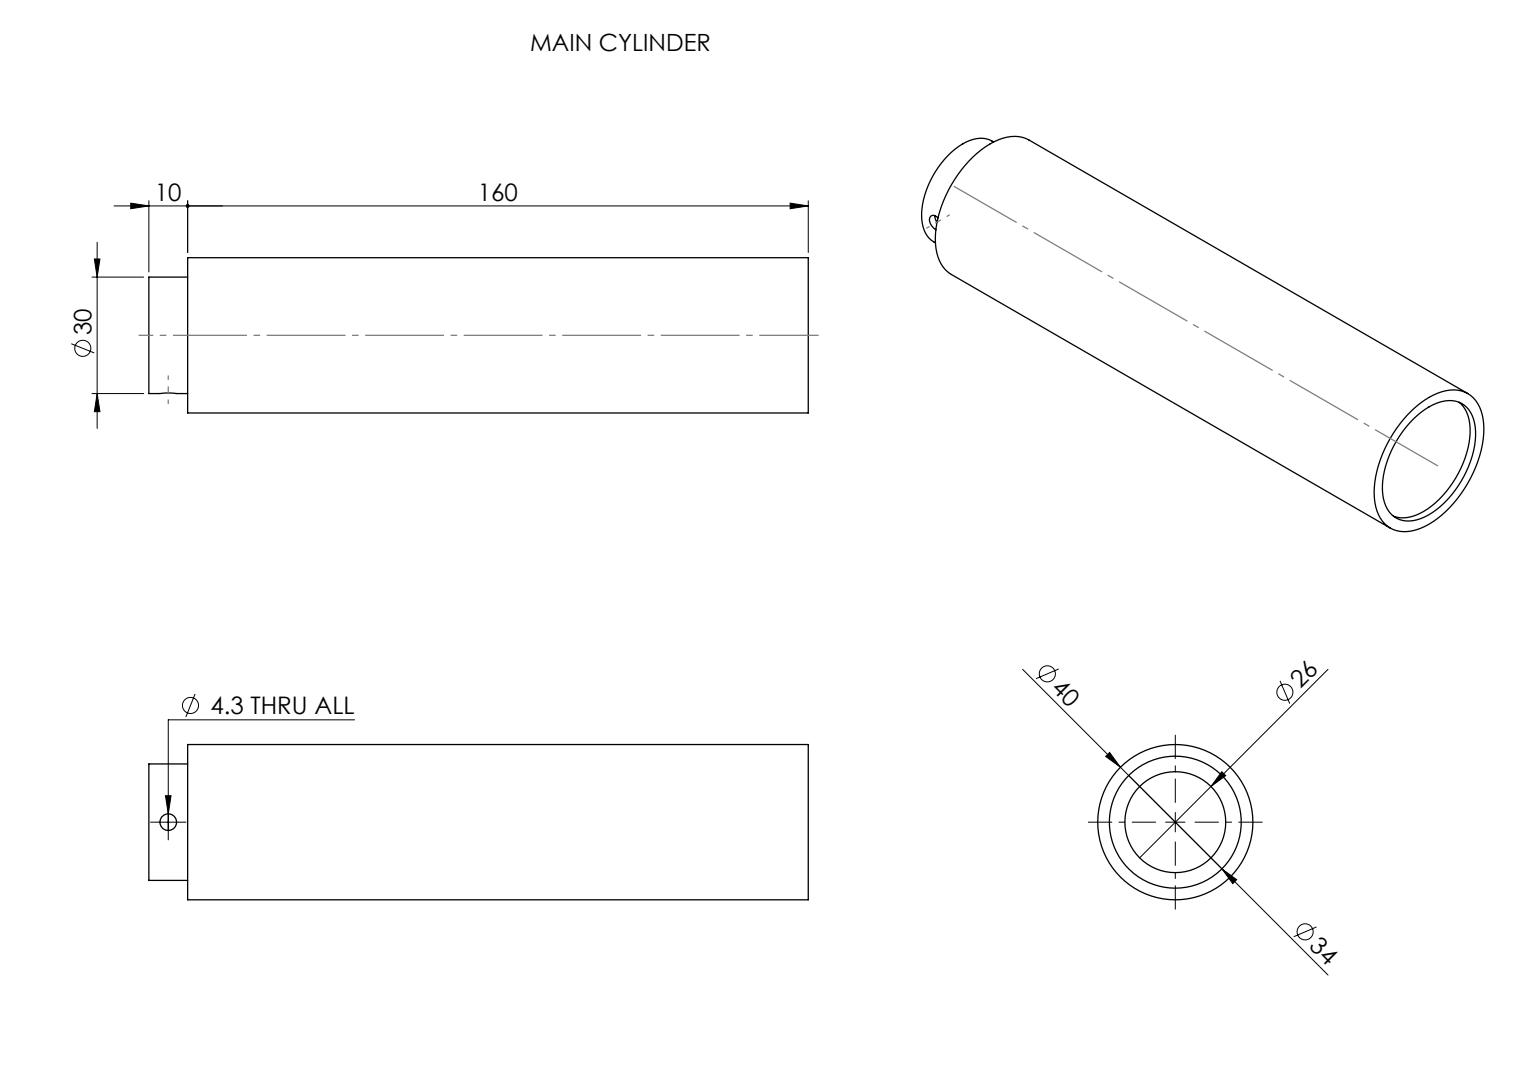
ISO-10303-21;
HEADER;
FILE_DESCRIPTION (('STEP AP214'),
    '1' );
FILE_NAME ('main cylinder.step',
    '2026-10-08T13:22:57',
    ( '' ),
    ( '' ),
    'SwSTEP 2.0',
    'SolidWorks 2026',
    '' );
FILE_SCHEMA (( 'AUTOMOTIVE_DESIGN' ));
ENDSEC;

DATA;
#66=DIRECTION ( 'NONE',  ( 1.000000000000000000, 4.755747939841215952E-17, -0.000000000000000000 ) ) ;
#75=CARTESIAN_POINT ( 'NONE',  ( -163.1352118936811451, 1.079191317860220156, 12.95565487998667820 ) ) ;
#78=ORIENTED_EDGE ( 'NONE', *, *, #9774, .F. ) ;
#81=DIRECTION ( 'NONE',  ( -4.755747939841216568E-17, 1.000000000000000000, 0.000000000000000000 ) ) ;
#98=CARTESIAN_POINT ( 'NONE',  ( -160.0000000000000284, 19.99999999999999289, 0.000000000000000000 ) ) ;
#120=CARTESIAN_POINT ( 'NONE',  ( -167.0926989554971556, -0.5670040589733402747, 14.99151548021192148 ) ) ;
#123=CARTESIAN_POINT ( 'NONE',  ( -166.9317395015584680, 0.9543248124665052456, 12.96558013998003922 ) ) ;
#132=ADVANCED_FACE ( 'NONE', ( #2160 ), #9918, .F. ) ;
#170=CARTESIAN_POINT ( 'NONE',  ( -165.9524913265358350, -1.932636693197999911, 14.87507538773749438 ) ) ;
#175=CARTESIAN_POINT ( 'NONE',  ( -166.3219090446497432, 1.718560695228406932, 12.88744630017030168 ) ) ;
#222=CARTESIAN_POINT ( 'NONE',  ( -8.084771497730057628E-16, 16.99999999999997868, 0.000000000000000000 ) ) ;
#225=CARTESIAN_POINT ( 'NONE',  ( -164.3051146695663363, -2.039487319166105372, 14.86080315614530534 ) ) ;
#228=CARTESIAN_POINT ( 'NONE',  ( -164.8603154174794270, 2.150053139255677870, 12.82096999065581322 ) ) ;
#239=DIRECTION ( 'NONE',  ( -4.755747939841215952E-17, 1.000000000000000000, 0.000000000000000000 ) ) ;
#245=CARTESIAN_POINT ( 'NONE',  ( 0.000000000000000000, 0.000000000000000000, 0.000000000000000000 ) ) ;
#257=APPLICATION_CONTEXT ( 'automotive_design' ) ;
#261=EDGE_LOOP ( 'NONE', ( #862, #304 ) ) ;
#274=DIRECTION ( 'NONE',  ( 0.000000000000000000, 1.000000000000000000, 0.000000000000000000 ) ) ;
#277=CARTESIAN_POINT ( 'NONE',  ( -164.4415472335243180, -2.080930162503950687, 14.85498226103907626 ) ) ;
#291=FACE_BOUND ( 'NONE', #7704, .T. ) ;
#297=DIRECTION ( 'NONE',  ( 1.000000000000000000, 4.755747939841215952E-17, -0.000000000000000000 ) ) ;
#302=ORIENTED_EDGE ( 'NONE', *, *, #7014, .T. ) ;
#304=ORIENTED_EDGE ( 'NONE', *, *, #4917, .T. ) ;
#308=PRODUCT ( 'main cylinder', 'main cylinder', '', ( #3194 ) ) ;
#311=ORIENTED_EDGE ( 'NONE', *, *, #4917, .F. ) ;
#314=DIRECTION ( 'NONE',  ( 0.000000000000000000, 1.000000000000000000, 0.000000000000000000 ) ) ;
#326=CARTESIAN_POINT ( 'NONE',  ( -164.0447505768503618, -1.931287831231678132, 14.87525146959452371 ) ) ;
#335=EDGE_LOOP ( 'NONE', ( #1912, #1497, #4062, #8563 ) ) ;
#345=VECTOR ( 'NONE', #3233, 1000.000000000000000 ) ;
#349=( NAMED_UNIT ( * ) SI_UNIT ( $, .STERADIAN. ) SOLID_ANGLE_UNIT ( ) );
#386=VECTOR ( 'NONE', #1036, 1000.000000000000000 ) ;
#401=ADVANCED_FACE ( 'NONE', ( #10107 ), #1214, .F. ) ;
#434=CARTESIAN_POINT ( 'NONE',  ( -162.8500000000000512, -5.808233104102145682E-15, 0.000000000000000000 ) ) ;
#443=FILL_AREA_STYLE ('',( #9851 ) ) ;
#468=DIRECTION ( 'NONE',  ( 1.000000000000000000, 4.755747939841215952E-17, -0.000000000000000000 ) ) ;
#485=ORIENTED_EDGE ( 'NONE', *, *, #7973, .F. ) ;
#507=MECHANICAL_DESIGN_GEOMETRIC_PRESENTATION_REPRESENTATION('',(#4963),#2980);
#517=ORIENTED_EDGE ( 'NONE', *, *, #4719, .F. ) ;
#544=CARTESIAN_POINT ( 'NONE',  ( -2.000000000000000888, -18.00000000000000355, 2.204364238465235822E-15 ) ) ;
#557=VERTEX_POINT ( 'NONE', #5547 ) ;
#594=VERTEX_POINT ( 'NONE', #10205 ) ;
#639=DIRECTION ( 'NONE',  ( 4.755747939841215952E-17, -1.000000000000000000, 0.000000000000000000 ) ) ;
#647=ORIENTED_EDGE ( 'NONE', *, *, #769, .T. ) ;
#664=EDGE_LOOP ( 'NONE', ( #485, #1187 ) ) ;
#675=AXIS2_PLACEMENT_3D ( 'NONE', #8769, #866, #81 ) ;
#679=CIRCLE ( 'NONE', #4292, 15.00000000000000000 ) ;
#699=CARTESIAN_POINT ( 'NONE',  ( -166.0761157388880918, -1.866610437352971719, 12.86553408738820714 ) ) ;
#714=DIRECTION ( 'NONE',  ( 1.000000000000000000, 4.755747939841215952E-17, -0.000000000000000000 ) ) ;
#715=ORIENTED_EDGE ( 'NONE', *, *, #7105, .T. ) ;
#755=EDGE_CURVE ( 'NONE', #7104, #6156, #3859, .T. ) ;
#769=EDGE_CURVE ( 'NONE', #9409, #594, #5277, .T. ) ;
#789=SHAPE_REPRESENTATION ( 'main cylinder', ( #3995 ), #10094 ) ;
#792=CARTESIAN_POINT ( 'NONE',  ( -166.4202771397491176, -1.620148664718404685, 12.89903195109847545 ) ) ;
#810=CARTESIAN_POINT ( 'NONE',  ( 0.000000000000000000, 5.592146987065130084E-32, 0.000000000000000000 ) ) ;
#812=CARTESIAN_POINT ( 'NONE',  ( -170.0000000000000284, -13.00000000000001066, 1.592040838891559687E-15 ) ) ;
#862=ORIENTED_EDGE ( 'NONE', *, *, #8540, .T. ) ;
#866=DIRECTION ( 'NONE',  ( 1.000000000000000000, 4.755747939841215952E-17, -0.000000000000000000 ) ) ;
#868=CIRCLE ( 'NONE', #8955, 18.00000000000000355 ) ;
#890=VECTOR ( 'NONE', #2246, 1000.000000000000000 ) ;
#913=VERTEX_POINT ( 'NONE', #98 ) ;
#955=CARTESIAN_POINT ( 'NONE',  ( -164.8564506259586153, -2.149904186608886381, 14.84513091884608649 ) ) ;
#970=PRODUCT_DEFINITION_FORMATION_WITH_SPECIFIED_SOURCE ( 'ANY', '', #308, .NOT_KNOWN. ) ;
#1003=CARTESIAN_POINT ( 'NONE',  ( -163.1340397805202542, -1.077317138390382345, 14.96172600814708353 ) ) ;
#1005=AXIS2_PLACEMENT_3D ( 'NONE', #7687, #7878, #1431 ) ;
#1035=VERTEX_POINT ( 'NONE', #4037 ) ;
#1036=DIRECTION ( 'NONE',  ( 1.000000000000000000, 4.755747939841215952E-17, -0.000000000000000000 ) ) ;
#1064=CARTESIAN_POINT ( 'NONE',  ( -162.8500000000000512, -5.808233196467851957E-15, 13.00000000000000178 ) ) ;
#1109=CARTESIAN_POINT ( 'NONE',  ( -165.5555415711045839, -2.081714733226260439, 14.85487199390593283 ) ) ;
#1131=EDGE_LOOP ( 'NONE', ( #4189, #4952 ) ) ;
#1146=ADVANCED_FACE ( 'NONE', ( #3187 ), #8668, .F. ) ;
#1156=CARTESIAN_POINT ( 'NONE',  ( -163.9215233434256618, 1.865203048549891163, 14.88378837804381583 ) ) ;
#1172=( LENGTH_UNIT ( ) NAMED_UNIT ( * ) SI_UNIT ( .MILLI., .METRE. ) );
#1180=AXIS2_PLACEMENT_3D ( 'NONE', #4946, #297, #8301 ) ;
#1187=ORIENTED_EDGE ( 'NONE', *, *, #8517, .F. ) ;
#1193=CARTESIAN_POINT ( 'NONE',  ( -160.0000000000000284, -7.609196703745946707E-15, 0.000000000000000000 ) ) ;
#1214=CYLINDRICAL_SURFACE ( 'NONE', #2628, 13.00000000000000178 ) ;
#1252=DIRECTION ( 'NONE',  ( -4.818676322157796389E-17, 1.000000000000000000, 0.000000000000000000 ) ) ;
#1259=CYLINDRICAL_SURFACE ( 'NONE', #4163, 15.00000000000000000 ) ;
#1306=CARTESIAN_POINT ( 'NONE',  ( -163.0677270160816192, 0.9532360713981521405, 14.97024790547416373 ) ) ;
#1330=FACE_BOUND ( 'NONE', #2547, .T. ) ;
#1341=AXIS2_PLACEMENT_3D ( 'NONE', #3965, #8237, #9078 ) ;
#1343=EDGE_CURVE ( 'NONE', #8824, #4150, #5768, .T. ) ;
#1345=ORIENTED_EDGE ( 'NONE', *, *, #5402, .F. ) ;
#1364=CARTESIAN_POINT ( 'NONE',  ( -164.8566404013504041, -2.149912913094245148, 12.82099350572476837 ) ) ;
#1399=VECTOR ( 'NONE', #8490, 1000.000000000000000 ) ;
#1400=EDGE_LOOP ( 'NONE', ( #5003, #9129, #5622, #9488 ) ) ;
#1431=DIRECTION ( 'NONE',  ( -4.755747939841215952E-17, 1.000000000000000000, 0.000000000000000000 ) ) ;
#1436=VERTEX_POINT ( 'NONE', #7998 ) ;
#1451=ORIENTED_EDGE ( 'NONE', *, *, #7973, .T. ) ;
#1468=CARTESIAN_POINT ( 'NONE',  ( -165.1407354622004391, -2.150086286197278707, 12.82096443211790060 ) ) ;
#1472=ORIENTED_EDGE ( 'NONE', *, *, #9157, .F. ) ;
#1497=ORIENTED_EDGE ( 'NONE', *, *, #1343, .F. ) ;
#1513=ORIENTED_EDGE ( 'NONE', *, *, #7634, .T. ) ;
#1521=CARTESIAN_POINT ( 'NONE',  ( -163.0673332015201709, -0.9523206289711777517, 12.96571997834879397 ) ) ;
#1565=ORIENTED_EDGE ( 'NONE', *, *, #2537, .F. ) ;
#1573=CARTESIAN_POINT ( 'NONE',  ( -163.3797476145753365, -1.420181920198508418, 12.92257903765585247 ) ) ;
#1586=CARTESIAN_POINT ( 'NONE',  ( -158.0000000000000284, -7.514081744949122117E-15, 0.000000000000000000 ) ) ;
#1596=SHAPE_DEFINITION_REPRESENTATION ( #1956, #789 ) ;
#1631=DIRECTION ( 'NONE',  ( 1.000000000000000000, 4.755747939841215952E-17, -0.000000000000000000 ) ) ;
#1663=ORIENTED_EDGE ( 'NONE', *, *, #6058, .F. ) ;
#1680=( GEOMETRIC_REPRESENTATION_CONTEXT ( 3 ) GLOBAL_UNCERTAINTY_ASSIGNED_CONTEXT ( ( #7319 ) ) GLOBAL_UNIT_ASSIGNED_CONTEXT ( ( #1172, #8987, #349 ) ) REPRESENTATION_CONTEXT ( 'NONE', 'WORKASPACE' ) );
#1687=CARTESIAN_POINT ( 'NONE',  ( -165.5651189253971722, 2.093213258176506386, 12.83083170865760181 ) ) ;
#1707=ORIENTED_EDGE ( 'NONE', *, *, #6644, .F. ) ;
#1716=AXIS2_PLACEMENT_3D ( 'NONE', #7873, #7733, #6362 ) ;
#1725=CIRCLE ( 'NONE', #5513, 13.00000000000000000 ) ;
#1731=CARTESIAN_POINT ( 'NONE',  ( -165.2804454449952516, -2.136238053246409141, 14.84712918936600623 ) ) ;
#1734=CARTESIAN_POINT ( 'NONE',  ( -160.0000000000000284, -7.609196703745946707E-15, 0.000000000000000000 ) ) ;
#1754=DIRECTION ( 'NONE',  ( 1.000000000000000000, 4.755747939841215952E-17, -0.000000000000000000 ) ) ;
#1760=ORIENTED_EDGE ( 'NONE', *, *, #4876, .T. ) ;
#1768=DIRECTION ( 'NONE',  ( -1.000000000000000000, -4.755747939841215952E-17, 0.000000000000000000 ) ) ;
#1779=DIRECTION ( 'NONE',  ( 0.000000000000000000, 1.000000000000000000, 0.000000000000000000 ) ) ;
#1784=ORIENTED_EDGE ( 'NONE', *, *, #755, .F. ) ;
#1789=DIRECTION ( 'NONE',  ( 1.000000000000000000, 4.755747939841215952E-17, -0.000000000000000000 ) ) ;
#1812=CYLINDRICAL_SURFACE ( 'NONE', #2046, 13.00000000000000178 ) ;
#1839=( LENGTH_UNIT ( ) NAMED_UNIT ( * ) SI_UNIT ( .MILLI., .METRE. ) );
#1844=UNCERTAINTY_MEASURE_WITH_UNIT (LENGTH_MEASURE( 1.000000000000000082E-05 ), #1839, 'distance_accuracy_value', 'NONE');
#1847=FILL_AREA_STYLE ('',( #5710 ) ) ;
#1882=CARTESIAN_POINT ( 'NONE',  ( -167.1500000000000341, -1.102909754258692077E-14, 15.00000000000000000 ) ) ;
#1885=CARTESIAN_POINT ( 'NONE',  ( -170.0000000000000284, 14.99999999999999289, 0.000000000000000000 ) ) ;
#1912=ORIENTED_EDGE ( 'NONE', *, *, #4905, .F. ) ;
#1918=DIRECTION ( 'NONE',  ( -5.102127870520027391E-17, 1.000000000000000000, 0.000000000000000000 ) ) ;
#1956=PRODUCT_DEFINITION_SHAPE ( 'NONE', 'NONE',  #4671 ) ;
#1979=CARTESIAN_POINT ( 'NONE',  ( -162.8500000000000512, -5.808233151972152598E-15, 15.00000000000000000 ) ) ;
#1987=DIRECTION ( 'NONE',  ( 1.000000000000000000, 4.755747939841215952E-17, -0.000000000000000000 ) ) ;
#1989=SURFACE_STYLE_FILL_AREA ( #443 ) ;
#1997=EDGE_CURVE ( 'NONE', #5632, #3401, #5774, .T. ) ;
#2038=PLANE ( 'NONE',  #5285 ) ;
#2041=UNCERTAINTY_MEASURE_WITH_UNIT (LENGTH_MEASURE( 1.000000000000000082E-05 ), #9661, 'distance_accuracy_value', 'NONE');
#2046=AXIS2_PLACEMENT_3D ( 'NONE', #8898, #2536, #8744 ) ;
#2074=EDGE_LOOP ( 'NONE', ( #5257, #2621, #7678, #7409 ) ) ;
#2081=CARTESIAN_POINT ( 'NONE',  ( -164.0471552234704689, 1.932476761857848668, 14.87509648533473516 ) ) ;
#2093=EDGE_CURVE ( 'NONE', #8307, #2751, #9346, .T. ) ;
#2106=FACE_OUTER_BOUND ( 'NONE', #8841, .T. ) ;
#2135=CARTESIAN_POINT ( 'NONE',  ( -165.6926619388180484, -2.040225341766198408, 12.83902055342544379 ) ) ;
#2158=ORIENTED_EDGE ( 'NONE', *, *, #7634, .F. ) ;
#2160=FACE_OUTER_BOUND ( 'NONE', #6889, .T. ) ;
#2171=EDGE_CURVE ( 'NONE', #6156, #1436, #3387, .T. ) ;
#2177=ORIENTED_EDGE ( 'NONE', *, *, #4861, .T. ) ;
#2192=CARTESIAN_POINT ( 'NONE',  ( -167.1500000000000341, -0.1422832181819098096, 13.00000000000000178 ) ) ;
#2246=DIRECTION ( 'NONE',  ( 1.000000000000000000, 4.755747939841215952E-17, -0.000000000000000000 ) ) ;
#2268=AXIS2_PLACEMENT_3D ( 'NONE', #2992, #6135, #9311 ) ;
#2292=CARTESIAN_POINT ( 'NONE',  ( -167.0388786721946701, -0.6964701277567462157, 12.98197609665553287 ) ) ;
#2298=CARTESIAN_POINT ( 'NONE',  ( 0.000000000000000000, 5.592146987065130084E-32, 0.000000000000000000 ) ) ;
#2312=DIRECTION ( 'NONE',  ( 0.000000000000000000, 1.000000000000000000, 0.000000000000000000 ) ) ;
#2340=CARTESIAN_POINT ( 'NONE',  ( -164.4413679183172121, -2.080883175690475539, 12.83240817167530246 ) ) ;
#2381=B_SPLINE_CURVE_WITH_KNOTS ( 'NONE', 3,
 ( #7253, #8759, #9543, #7306, #8820, #123, #4778, #3333, #2450, #175, #4058, #1687, #3228, #228, #6470, #9648, #5550, #3381, #8709, #5596, #5744, #4829, #7982, #75, #8079, #9693, #4205, #4157, #8913, #1064 ),
 .UNSPECIFIED., .F., .F.,
 ( 4, 2, 2, 2, 2, 2, 2, 2, 2, 2, 2, 2, 2, 2, 4 ),
 ( 5.712404575677604335E-19, 0.0004208408401708223071, 0.0008416816803416437469, 0.001262522520512465458, 0.001683363360683286626, 0.002525045041024870634, 0.003366726721366455292, 0.003787567561537246753, 0.004208408401708039516, 0.004629249241878830544, 0.005050090082049622439, 0.005470930922220414334, 0.005891771762391206230, 0.006312612602561998125, 0.006733453442732789153 ),
 .UNSPECIFIED. ) ;
#2402=CYLINDRICAL_SURFACE ( 'NONE', #8419, 18.00000000000000355 ) ;
#2450=CARTESIAN_POINT ( 'NONE',  ( -166.6189502573242578, 1.421653495296104408, 12.92241587668698166 ) ) ;
#2468=EDGE_LOOP ( 'NONE', ( #78, #6017, #4100, #7426 ) ) ;
#2470=LINE ( 'NONE', #5570, #8453 ) ;
#2499=CARTESIAN_POINT ( 'NONE',  ( -166.7173525949050088, -1.323475700837307700, 14.94282300546550069 ) ) ;
#2504=AXIS2_PLACEMENT_3D ( 'NONE', #2298, #2959, #5442 ) ;
#2507=EDGE_LOOP ( 'NONE', ( #9847, #7329 ) ) ;
#2532=ORIENTED_EDGE ( 'NONE', *, *, #8210, .F. ) ;
#2536=DIRECTION ( 'NONE',  ( 1.000000000000000000, 4.755747939841215952E-17, -0.000000000000000000 ) ) ;
#2537=EDGE_CURVE ( 'NONE', #594, #9409, #5452, .T. ) ;
#2547=EDGE_LOOP ( 'NONE', ( #3091, #8288 ) ) ;
#2551=CARTESIAN_POINT ( 'NONE',  ( -165.1406648078596220, -2.150094845865166082, 14.84510330590739180 ) ) ;
#2569=SURFACE_SIDE_STYLE ('',( #6482 ) ) ;
#2579=ADVANCED_FACE ( 'NONE', ( #5084 ), #8235, .T. ) ;
#2621=ORIENTED_EDGE ( 'NONE', *, *, #8540, .F. ) ;
#2628=AXIS2_PLACEMENT_3D ( 'NONE', #6162, #6212, #9540 ) ;
#2638=VECTOR ( 'NONE', #5736, 1000.000000000000000 ) ;
#2644=CARTESIAN_POINT ( 'NONE',  ( -162.9064615436232373, -0.5639517720651365806, 14.99163496215254199 ) ) ;
#2650=CARTESIAN_POINT ( 'NONE',  ( -162.8500000000000227, 0.1404123523451087929, 14.99999999999999822 ) ) ;
#2653=AXIS2_PLACEMENT_3D ( 'NONE', #3032, #6790, #2312 ) ;
#2689=CARTESIAN_POINT ( 'NONE',  ( 9.511495879682431411E-16, -20.00000000000000000, 2.449293598294706513E-15 ) ) ;
#2702=DIRECTION ( 'NONE',  ( -0.000000000000000000, -0.000000000000000000, -1.000000000000000000 ) ) ;
#2746=CARTESIAN_POINT ( 'NONE',  ( -163.6887781248447880, 1.709617356372435948, 14.90246111853683608 ) ) ;
#2751=VERTEX_POINT ( 'NONE', #3851 ) ;
#2753=DIRECTION ( 'NONE',  ( -4.755747939841215952E-17, 1.000000000000000000, 0.000000000000000000 ) ) ;
#2784=CARTESIAN_POINT ( 'NONE',  ( 0.000000000000000000, 0.000000000000000000, 0.000000000000000000 ) ) ;
#2796=CARTESIAN_POINT ( 'NONE',  ( -164.8603691185176388, 2.150052187497858647, 14.84510948406350472 ) ) ;
#2802=AXIS2_PLACEMENT_3D ( 'NONE', #5191, #5142, #5952 ) ;
#2807=DIRECTION ( 'NONE',  ( 1.000000000000000000, 4.755747939841215952E-17, -0.000000000000000000 ) ) ;
#2809=FACE_OUTER_BOUND ( 'NONE', #4327, .T. ) ;
#2840=DIRECTION ( 'NONE',  ( 0.000000000000000000, 1.000000000000000000, 0.000000000000000000 ) ) ;
#2858=FACE_OUTER_BOUND ( 'NONE', #6255, .T. ) ;
#2900=CARTESIAN_POINT ( 'NONE',  ( -166.3099971560734218, -1.710604296556395898, 12.88720430579052767 ) ) ;
#2921=ORIENTED_EDGE ( 'NONE', *, *, #8517, .T. ) ;
#2922=EDGE_CURVE ( 'NONE', #3401, #5632, #5460, .T. ) ;
#2925=PLANE ( 'NONE',  #2986 ) ;
#2959=DIRECTION ( 'NONE',  ( 1.000000000000000000, 4.755747939841215952E-17, -0.000000000000000000 ) ) ;
#2980=( GEOMETRIC_REPRESENTATION_CONTEXT ( 3 ) GLOBAL_UNCERTAINTY_ASSIGNED_CONTEXT ( ( #1844 ) ) GLOBAL_UNIT_ASSIGNED_CONTEXT ( ( #1839, #5753, #6718 ) ) REPRESENTATION_CONTEXT ( 'NONE', 'WORKASPACE' ) );
#2986=AXIS2_PLACEMENT_3D ( 'NONE', #5250, #4487, #7641 ) ;
#2992=CARTESIAN_POINT ( 'NONE',  ( -165.0000000000000284, -6.071532165918824830E-15, 0.000000000000000000 ) ) ;
#3009=CARTESIAN_POINT ( 'NONE',  ( -164.7162546839571462, -2.135798021625797460, 12.82338259142922432 ) ) ;
#3032=CARTESIAN_POINT ( 'NONE',  ( -170.0000000000000284, -8.084771497730068080E-15, 0.000000000000000000 ) ) ;
#3059=FACE_BOUND ( 'NONE', #8461, .T. ) ;
#3091=ORIENTED_EDGE ( 'NONE', *, *, #3345, .T. ) ;
#3108=CARTESIAN_POINT ( 'NONE',  ( 0.000000000000000000, 20.00000000000000000, 0.000000000000000000 ) ) ;
#3118=DIRECTION ( 'NONE',  ( 1.000000000000000000, 4.755747939841215952E-17, -0.000000000000000000 ) ) ;
#3124=DIRECTION ( 'NONE',  ( 0.000000000000000000, 1.000000000000000000, 0.000000000000000000 ) ) ;
#3160=LINE ( 'NONE', #6249, #1399 ) ;
#3187=FACE_OUTER_BOUND ( 'NONE', #2468, .T. ) ;
#3188=DIRECTION ( 'NONE',  ( 0.000000000000000000, 1.000000000000000000, 0.000000000000000000 ) ) ;
#3194=PRODUCT_CONTEXT ( 'NONE', #7122, 'mechanical' ) ;
#3228=CARTESIAN_POINT ( 'NONE',  ( -165.2818157524650360, 2.149893257473834307, 12.82099680185394242 ) ) ;
#3233=DIRECTION ( 'NONE',  ( -0.000000000000000000, -0.000000000000000000, -1.000000000000000000 ) ) ;
#3320=AXIS2_PLACEMENT_3D ( 'NONE', #1193, #3613, #2840 ) ;
#3324=EDGE_CURVE ( 'NONE', #4862, #6875, #7042, .T. ) ;
#3327=COLOUR_RGB ( '', 0.72549020, 0.75294118, 0.79215686) ;
#3330=CARTESIAN_POINT ( 'NONE',  ( -162.8500000000000512, -5.808233151972152598E-15, 15.00000000000000000 ) ) ;
#3333=CARTESIAN_POINT ( 'NONE',  ( -166.7096159853958568, 1.311273010886724544, 12.93423035082597927 ) ) ;
#3345=EDGE_CURVE ( 'NONE', #2751, #5081, #9369, .T. ) ;
#3381=CARTESIAN_POINT ( 'NONE',  ( -164.0468713975789115, 1.932340315393523023, 12.85570084551372183 ) ) ;
#3387=LINE ( 'NONE', #6568, #345 ) ;
#3401=VERTEX_POINT ( 'NONE', #222 ) ;
#3402=CARTESIAN_POINT ( 'NONE',  ( -2.000000000000001776, -9.511495879682425741E-17, 0.000000000000000000 ) ) ;
#3415=AXIS2_PLACEMENT_3D ( 'NONE', #7350, #5645, #7150 ) ;
#3434=SURFACE_STYLE_USAGE ( .BOTH. , #8922 ) ;
#3454=ORIENTED_EDGE ( 'NONE', *, *, #4219, .F. ) ;
#3479=CARTESIAN_POINT ( 'NONE',  ( -167.0398489105598685, 0.6938099590080268886, 14.98451262434803688 ) ) ;
#3486=VERTEX_POINT ( 'NONE', #4612 ) ;
#3488=CARTESIAN_POINT ( 'NONE',  ( 0.000000000000000000, 4.523427693460793966E-32, 0.000000000000000000 ) ) ;
#3613=DIRECTION ( 'NONE',  ( 1.000000000000000000, 4.755747939841215952E-17, -0.000000000000000000 ) ) ;
#3634=VECTOR ( 'NONE', #8122, 1000.000000000000000 ) ;
#3643=CIRCLE ( 'NONE', #2653, 15.00000000000000178 ) ;
#3652=CARTESIAN_POINT ( 'NONE',  ( -165.0000000000000284, -6.071532165918824830E-15, 0.000000000000000000 ) ) ;
#3676=AXIS2_PLACEMENT_3D ( 'NONE', #3108, #7719, #639 ) ;
#3681=CARTESIAN_POINT ( 'NONE',  ( 8.084771497730057628E-16, -16.99999999999997868, 2.081899558550498307E-15 ) ) ;
#3685=CARTESIAN_POINT ( 'NONE',  ( -162.9598814269480158, 0.6930036797044089036, 14.98454961815950170 ) ) ;
#3714=EDGE_LOOP ( 'NONE', ( #6183, #10124 ) ) ;
#3731=FACE_BOUND ( 'NONE', #1131, .T. ) ;
#3846=DIRECTION ( 'NONE',  ( 0.000000000000000000, 1.000000000000000000, 0.000000000000000000 ) ) ;
#3851=CARTESIAN_POINT ( 'NONE',  ( -160.0000000000000284, 14.99999999999999289, 0.000000000000000000 ) ) ;
#3857=FACE_OUTER_BOUND ( 'NONE', #6839, .T. ) ;
#3859=B_SPLINE_CURVE_WITH_KNOTS ( 'NONE', 3,
 ( #3330, #5741, #2644, #8910, #1003, #5795, #6511, #9645, #4929, #7402, #326, #225, #277, #8969, #955, #2551, #1731, #1109, #8127, #170, #4980, #5030, #6466, #2499, #4105, #120, #7354, #1882 ),
 .UNSPECIFIED., .F., .F.,
 ( 4, 2, 2, 2, 2, 2, 2, 2, 2, 2, 2, 2, 2, 4 ),
 ( 0.006730547602530746569, 0.007571661104541401940, 0.007992217855546712713, 0.008412774606552025219, 0.008833331357557337726, 0.009253888108562648498, 0.009674444859567959271, 0.01009500161057327178, 0.01051555836157858255, 0.01093611511258389332, 0.01135667186358920583, 0.01177722861459451487, 0.01261834211660513988, 0.01345945561861576142 ),
 .UNSPECIFIED. ) ;
#3871=ADVANCED_FACE ( 'NONE', ( #9206, #7705 ), #3877, .F. ) ;
#3877=PLANE ( 'NONE',  #8542 ) ;
#3895=ADVANCED_FACE ( 'NONE', ( #6854 ), #9411, .F. ) ;
#3905=CYLINDRICAL_SURFACE ( 'NONE', #1005, 20.00000000000000000 ) ;
#3911=AXIS2_PLACEMENT_3D ( 'NONE', #4877, #66, #274 ) ;
#3953=CYLINDRICAL_SURFACE ( 'NONE', #6266, 18.00000000000000355 ) ;
#3962=CARTESIAN_POINT ( 'NONE',  ( -7.133621909761823559E-16, 15.00000000000000000, 0.000000000000000000 ) ) ;
#3963=ORIENTED_EDGE ( 'NONE', *, *, #9284, .T. ) ;
#3965=CARTESIAN_POINT ( 'NONE',  ( -160.0000000000000284, -7.609196703745946707E-15, 0.000000000000000000 ) ) ;
#3969=AXIS2_PLACEMENT_3D ( 'NONE', #4154, #8817, #4880 ) ;
#3971=CIRCLE ( 'NONE', #9752, 18.00000000000000355 ) ;
#3987=CIRCLE ( 'NONE', #4973, 15.00000000000000178 ) ;
#3989=ORIENTED_EDGE ( 'NONE', *, *, #4905, .T. ) ;
#3995=AXIS2_PLACEMENT_3D ( 'NONE', #245, #8930, #7419 ) ;
#4009=DIRECTION ( 'NONE',  ( -4.755747939841215952E-17, 1.000000000000000000, 0.000000000000000000 ) ) ;
#4037=CARTESIAN_POINT ( 'NONE',  ( -2.000000000000000888, -16.99999999999997868, 2.081899558550498307E-15 ) ) ;
#4058=CARTESIAN_POINT ( 'NONE',  ( -166.0823889414796497, 1.878652528652014819, 12.86399816373932126 ) ) ;
#4062=ORIENTED_EDGE ( 'NONE', *, *, #8698, .T. ) ;
#4085=VERTEX_POINT ( 'NONE', #8002 ) ;
#4100=ORIENTED_EDGE ( 'NONE', *, *, #9010, .T. ) ;
#4105=CARTESIAN_POINT ( 'NONE',  ( -166.8777055324365790, -1.084022349717994604, 14.96301859724961147 ) ) ;
#4108=CARTESIAN_POINT ( 'NONE',  ( 0.000000000000000000, 0.000000000000000000, 0.000000000000000000 ) ) ;
#4145=VECTOR ( 'NONE', #10032, 1000.000000000000000 ) ;
#4150=VERTEX_POINT ( 'NONE', #7227 ) ;
#4154=CARTESIAN_POINT ( 'NONE',  ( 0.000000000000000000, 4.523427693460793966E-32, 0.000000000000000000 ) ) ;
#4157=CARTESIAN_POINT ( 'NONE',  ( -162.8640792231055912, 0.2831181362186585004, 12.99765045411212938 ) ) ;
#4163=AXIS2_PLACEMENT_3D ( 'NONE', #4181, #2807, #4955 ) ;
#4181=CARTESIAN_POINT ( 'NONE',  ( 0.000000000000000000, 0.000000000000000000, 0.000000000000000000 ) ) ;
#4189=ORIENTED_EDGE ( 'NONE', *, *, #2922, .F. ) ;
#4205=CARTESIAN_POINT ( 'NONE',  ( -162.9192246874586374, 0.5591847127235903825, 12.98870223168555604 ) ) ;
#4213=DIRECTION ( 'NONE',  ( 1.000000000000000000, 4.755747939841215952E-17, -0.000000000000000000 ) ) ;
#4219=EDGE_CURVE ( 'NONE', #5716, #5081, #2470, .T. ) ;
#4220=SURFACE_STYLE_USAGE ( .BOTH. , #2569 ) ;
#4226=ORIENTED_EDGE ( 'NONE', *, *, #8698, .F. ) ;
#4256=CARTESIAN_POINT ( 'NONE',  ( -166.7097254823910077, 1.311132300232774162, 14.94304721624505028 ) ) ;
#4292=AXIS2_PLACEMENT_3D ( 'NONE', #1734, #8866, #1779 ) ;
#4317=CARTESIAN_POINT ( 'NONE',  ( -162.8500000000000512, -5.808233151972152598E-15, 15.00000000000000000 ) ) ;
#4327=EDGE_LOOP ( 'NONE', ( #9574, #5316 ) ) ;
#4329=ORIENTED_EDGE ( 'NONE', *, *, #8243, .F. ) ;
#4343=CARTESIAN_POINT ( 'NONE',  ( -2.000000000000001776, -9.511495879682425741E-17, 0.000000000000000000 ) ) ;
#4356=CARTESIAN_POINT ( 'NONE',  ( -2.000000000000001776, -9.511495879682425741E-17, 0.000000000000000000 ) ) ;
#4364=CARTESIAN_POINT ( 'NONE',  ( -158.0000000000000284, -7.514081744949122117E-15, 0.000000000000000000 ) ) ;
#4392=ADVANCED_FACE ( 'NONE', ( #9287, #2858 ), #1259, .T. ) ;
#4458=CARTESIAN_POINT ( 'NONE',  ( -166.8657786825345397, 1.077543057910302471, 14.96170541662921316 ) ) ;
#4478=CIRCLE ( 'NONE', #3320, 20.00000000000000000 ) ;
#4487=DIRECTION ( 'NONE',  ( 1.000000000000000000, 4.755747939841215952E-17, -0.000000000000000000 ) ) ;
#4588=DIRECTION ( 'NONE',  ( -4.755747939841216568E-17, 1.000000000000000000, 0.000000000000000000 ) ) ;
#4600=B_SPLINE_CURVE_WITH_KNOTS ( 'NONE', 3,
 ( #9378, #7037, #8650, #1521, #6252, #5492, #1573, #10041, #8440, #6099, #7819, #8545, #2340, #3009, #1364, #1468, #7865, #9431, #2135, #9278, #699, #2900, #792, #7724, #5435, #2292, #5279, #6820, #2192, #6044 ),
 .UNSPECIFIED., .F., .F.,
 ( 4, 2, 2, 2, 2, 2, 2, 2, 2, 2, 2, 2, 2, 2, 4 ),
 ( 0.006733453442732789153, 0.007574925429288498560, 0.007995661422566354565, 0.008416397415844208835, 0.008837133409122063105, 0.009257869402399917375, 0.009678605395677773379, 0.01009934138895562765, 0.01052007738223348365, 0.01094081337551133792, 0.01136154936878919219, 0.01178228536206704646, 0.01262375734862281572, 0.01304449334190071683, 0.01346522933517861620 ),
 .UNSPECIFIED. ) ;
#4602=CARTESIAN_POINT ( 'NONE',  ( -170.0000000000000284, 12.99999999999999289, 0.000000000000000000 ) ) ;
#4612=CARTESIAN_POINT ( 'NONE',  ( -158.0000000000000284, -13.00000000000000711, 1.592040838891559095E-15 ) ) ;
#4617=CARTESIAN_POINT ( 'NONE',  ( -170.0000000000000284, -8.084771497730068080E-15, 0.000000000000000000 ) ) ;
#4625=CARTESIAN_POINT ( 'NONE',  ( 8.560346291714190440E-16, -18.00000000000000355, 2.204364238465235822E-15 ) ) ;
#4640=AXIS2_PLACEMENT_3D ( 'NONE', #810, #5456, #4588 ) ;
#4643=CIRCLE ( 'NONE', #7281, 16.99999999999997868 ) ;
#4671=PRODUCT_DEFINITION ( 'UNKNOWN', '', #970, #6776 ) ;
#4673=ORIENTED_EDGE ( 'NONE', *, *, #2093, .F. ) ;
#4682=CARTESIAN_POINT ( 'NONE',  ( 0.000000000000000000, 0.000000000000000000, 0.000000000000000000 ) ) ;
#4719=EDGE_CURVE ( 'NONE', #4150, #8824, #868, .T. ) ;
#4778=CARTESIAN_POINT ( 'NONE',  ( -166.8656692072818828, 1.077730084761960194, 12.95578054544406044 ) ) ;
#4829=CARTESIAN_POINT ( 'NONE',  ( -163.3796219069818960, 1.420182798501361754, 12.92258649737903298 ) ) ;
#4839=CARTESIAN_POINT ( 'NONE',  ( -170.0000000000000284, -8.084771497730068080E-15, 0.000000000000000000 ) ) ;
#4861=EDGE_CURVE ( 'NONE', #7065, #3486, #7624, .T. ) ;
#4862=VERTEX_POINT ( 'NONE', #544 ) ;
#4876=EDGE_CURVE ( 'NONE', #557, #1035, #7975, .T. ) ;
#4877=CARTESIAN_POINT ( 'NONE',  ( -160.0000000000000284, -7.609196703745946707E-15, 0.000000000000000000 ) ) ;
#4880=DIRECTION ( 'NONE',  ( -4.755747939841215952E-17, 1.000000000000000000, 0.000000000000000000 ) ) ;
#4905=EDGE_CURVE ( 'NONE', #4150, #4862, #10106, .T. ) ;
#4917=EDGE_CURVE ( 'NONE', #7065, #6270, #6149, .T. ) ;
#4929=CARTESIAN_POINT ( 'NONE',  ( -163.6882045205299789, -1.709201878644992956, 14.90250977739813365 ) ) ;
#4946=CARTESIAN_POINT ( 'NONE',  ( 0.000000000000000000, 0.000000000000000000, 0.000000000000000000 ) ) ;
#4952=ORIENTED_EDGE ( 'NONE', *, *, #1997, .F. ) ;
#4955=DIRECTION ( 'NONE',  ( -4.755747939841215952E-17, 1.000000000000000000, 0.000000000000000000 ) ) ;
#4963=STYLED_ITEM ( 'NONE', ( #9754 ), #7117 ) ;
#4973=AXIS2_PLACEMENT_3D ( 'NONE', #4839, #1789, #3188 ) ;
#4980=CARTESIAN_POINT ( 'NONE',  ( -166.0759530565494231, -1.866699619213640027, 14.88360162420890020 ) ) ;
#5003=ORIENTED_EDGE ( 'NONE', *, *, #9284, .F. ) ;
#5030=CARTESIAN_POINT ( 'NONE',  ( -166.3097507274169686, -1.710787970585769813, 14.90232764692231271 ) ) ;
#5078=CARTESIAN_POINT ( 'NONE',  ( -166.0822128819447698, 1.878756849882351254, 14.88227075829311552 ) ) ;
#5081=VERTEX_POINT ( 'NONE', #8659 ) ;
#5084=FACE_OUTER_BOUND ( 'NONE', #9517, .T. ) ;
#5140=ORIENTED_EDGE ( 'NONE', *, *, #2171, .T. ) ;
#5142=DIRECTION ( 'NONE',  ( 1.000000000000000000, 4.755747939841215952E-17, -0.000000000000000000 ) ) ;
#5151=FACE_OUTER_BOUND ( 'NONE', #9603, .T. ) ;
#5185=CARTESIAN_POINT ( 'NONE',  ( -167.1360214673730979, 0.2820915794957485345, 14.99797831373487078 ) ) ;
#5191=CARTESIAN_POINT ( 'NONE',  ( 0.000000000000000000, 0.000000000000000000, 0.000000000000000000 ) ) ;
#5207=ORIENTED_EDGE ( 'NONE', *, *, #7105, .F. ) ;
#5229=CARTESIAN_POINT ( 'NONE',  ( -163.1351247077966491, 1.079043896566285632, 14.96159378939550599 ) ) ;
#5250=CARTESIAN_POINT ( 'NONE',  ( -160.0000000000000284, 14.99999999999999289, 0.000000000000000000 ) ) ;
#5257=ORIENTED_EDGE ( 'NONE', *, *, #4861, .F. ) ;
#5277=CIRCLE ( 'NONE', #3969, 20.00000000000000000 ) ;
#5279=CARTESIAN_POINT ( 'NONE',  ( -167.0804693905882914, -0.5605331060369084240, 12.98865281316615317 ) ) ;
#5282=ORIENTED_EDGE ( 'NONE', *, *, #8294, .F. ) ;
#5285=AXIS2_PLACEMENT_3D ( 'NONE', #7316, #4213, #239 ) ;
#5295=CARTESIAN_POINT ( 'NONE',  ( -160.0000000000000284, -20.00000000000000711, 2.449293598294706907E-15 ) ) ;
#5316=ORIENTED_EDGE ( 'NONE', *, *, #4719, .T. ) ;
#5339=DIRECTION ( 'NONE',  ( 1.000000000000000000, 4.755747939841215952E-17, -0.000000000000000000 ) ) ;
#5398=FACE_OUTER_BOUND ( 'NONE', #7953, .T. ) ;
#5402=EDGE_CURVE ( 'NONE', #913, #594, #6412, .T. ) ;
#5415=ORIENTED_EDGE ( 'NONE', *, *, #9157, .T. ) ;
#5435=CARTESIAN_POINT ( 'NONE',  ( -166.8775874622578783, -1.084229144011057411, 12.95729691005224637 ) ) ;
#5442=DIRECTION ( 'NONE',  ( -4.755747939841216568E-17, 1.000000000000000000, 0.000000000000000000 ) ) ;
#5452=CIRCLE ( 'NONE', #7102, 20.00000000000000000 ) ;
#5453=CIRCLE ( 'NONE', #7434, 13.00000000000000000 ) ;
#5456=DIRECTION ( 'NONE',  ( 1.000000000000000000, 4.755747939841215952E-17, -0.000000000000000000 ) ) ;
#5460=CIRCLE ( 'NONE', #2504, 16.99999999999997868 ) ;
#5492=CARTESIAN_POINT ( 'NONE',  ( -163.2909762424711460, -1.312104824217039889, 12.93415009021162554 ) ) ;
#5513=AXIS2_PLACEMENT_3D ( 'NONE', #7491, #468, #314 ) ;
#5539=LINE ( 'NONE', #8857, #3634 ) ;
#5547=CARTESIAN_POINT ( 'NONE',  ( -2.000000000000002665, 16.99999999999997868, 0.000000000000000000 ) ) ;
#5550=CARTESIAN_POINT ( 'NONE',  ( -164.3074826167014351, 2.040297258018446858, 12.83900971347711639 ) ) ;
#5570=CARTESIAN_POINT ( 'NONE',  ( 7.133621909761823559E-16, -15.00000000000000000, 1.836970198721029589E-15 ) ) ;
#5596=CARTESIAN_POINT ( 'NONE',  ( -163.6886816470472468, 1.709539868520255412, 12.88734415733343752 ) ) ;
#5622=ORIENTED_EDGE ( 'NONE', *, *, #1997, .T. ) ;
#5624=VECTOR ( 'NONE', #5833, 1000.000000000000000 ) ;
#5632=VERTEX_POINT ( 'NONE', #3681 ) ;
#5644=ORIENTED_EDGE ( 'NONE', *, *, #9435, .F. ) ;
#5645=DIRECTION ( 'NONE',  ( 1.000000000000000000, 4.755747939841215952E-17, -0.000000000000000000 ) ) ;
#5710=FILL_AREA_STYLE_COLOUR ( '', #3327 ) ;
#5716=VERTEX_POINT ( 'NONE', #6754 ) ;
#5736=DIRECTION ( 'NONE',  ( 1.000000000000000000, 4.755747939841215952E-17, -0.000000000000000000 ) ) ;
#5741=CARTESIAN_POINT ( 'NONE',  ( -162.8500000000000227, -0.2807562947469993686, 14.99999999999999822 ) ) ;
#5744=CARTESIAN_POINT ( 'NONE',  ( -163.5798452441948427, 1.620402670652003829, 12.89900989023366407 ) ) ;
#5753=( NAMED_UNIT ( * ) PLANE_ANGLE_UNIT ( ) SI_UNIT ( $, .RADIAN. ) );
#5768=CIRCLE ( 'NONE', #9421, 18.00000000000000355 ) ;
#5774=CIRCLE ( 'NONE', #4640, 16.99999999999997868 ) ;
#5775=VECTOR ( 'NONE', #2702, 1000.000000000000000 ) ;
#5795=CARTESIAN_POINT ( 'NONE',  ( -163.2908874445610365, -1.312003822475822146, 14.94297504947871325 ) ) ;
#5798=DIRECTION ( 'NONE',  ( 1.000000000000000000, 4.755747939841215952E-17, -0.000000000000000000 ) ) ;
#5799=CLOSED_SHELL ( 'NONE', ( #132, #9113, #7853, #4392, #401, #7617, #8610, #8088, #7234, #6359, #3871, #10214, #6977, #2579, #6225, #1146, #3895 ) ) ;
#5833=DIRECTION ( 'NONE',  ( 1.000000000000000000, 4.755747939841215952E-17, -0.000000000000000000 ) ) ;
#5843=CARTESIAN_POINT ( 'NONE',  ( -165.5648848242107647, 2.093279044514479992, 14.85361548801915887 ) ) ;
#5891=CARTESIAN_POINT ( 'NONE',  ( -163.3795937461757433, 1.420165590446639259, 14.93295938614575036 ) ) ;
#5945=CARTESIAN_POINT ( 'NONE',  ( -164.7177004374966032, 2.136022552468798796, 14.84716063139783593 ) ) ;
#5948=STYLED_ITEM ( 'NONE', ( #9762 ), #9686 ) ;
#5952=DIRECTION ( 'NONE',  ( -4.755747939841215952E-17, 1.000000000000000000, 0.000000000000000000 ) ) ;
#5962=SHAPE_REPRESENTATION_RELATIONSHIP ( 'NONE' , 'NONE' ,  #789, #9686 ) ;
#6001=DIRECTION ( 'NONE',  ( 1.000000000000000000, 4.755747939841215952E-17, -0.000000000000000000 ) ) ;
#6017=ORIENTED_EDGE ( 'NONE', *, *, #4876, .F. ) ;
#6035=ORIENTED_EDGE ( 'NONE', *, *, #769, .F. ) ;
#6044=CARTESIAN_POINT ( 'NONE',  ( -167.1500000000000341, -5.483569848023176209E-15, 13.00000000000000178 ) ) ;
#6058=EDGE_CURVE ( 'NONE', #6270, #4085, #3160, .T. ) ;
#6099=CARTESIAN_POINT ( 'NONE',  ( -163.9212390029829578, -1.865053163018561833, 12.86575946079389787 ) ) ;
#6135=DIRECTION ( 'NONE',  ( -0.000000000000000000, -0.000000000000000000, -1.000000000000000000 ) ) ;
#6144=VECTOR ( 'NONE', #9644, 1000.000000000000000 ) ;
#6149=CIRCLE ( 'NONE', #1716, 13.00000000000000178 ) ;
#6156=VERTEX_POINT ( 'NONE', #6980 ) ;
#6162=CARTESIAN_POINT ( 'NONE',  ( 0.000000000000000000, 0.000000000000000000, 0.000000000000000000 ) ) ;
#6183=ORIENTED_EDGE ( 'NONE', *, *, #7014, .F. ) ;
#6192=CARTESIAN_POINT ( 'NONE',  ( 8.084771497730057628E-16, -16.99999999999997868, 2.081899558550498307E-15 ) ) ;
#6203=FACE_OUTER_BOUND ( 'NONE', #7664, .T. ) ;
#6212=DIRECTION ( 'NONE',  ( 1.000000000000000000, 4.755747939841215952E-17, -0.000000000000000000 ) ) ;
#6225=ADVANCED_FACE ( 'NONE', ( #3731, #9425 ), #8591, .F. ) ;
#6234=DIRECTION ( 'NONE',  ( -4.755747939841215952E-17, 1.000000000000000000, 0.000000000000000000 ) ) ;
#6249=CARTESIAN_POINT ( 'NONE',  ( -6.182472321793581601E-16, 13.00000000000000178, 0.000000000000000000 ) ) ;
#6252=CARTESIAN_POINT ( 'NONE',  ( -163.1342507503006232, -1.077664609596973300, 12.95579008069663551 ) ) ;
#6255=EDGE_LOOP ( 'NONE', ( #302, #9622, #8000, #4673 ) ) ;
#6259=DIRECTION ( 'NONE',  ( -5.102127870520027391E-17, 1.000000000000000000, 0.000000000000000000 ) ) ;
#6266=AXIS2_PLACEMENT_3D ( 'NONE', #4682, #6998, #10111 ) ;
#6267=AXIS2_PLACEMENT_3D ( 'NONE', #8699, #1768, #9637 ) ;
#6270=VERTEX_POINT ( 'NONE', #9730 ) ;
#6291=AXIS2_PLACEMENT_3D ( 'NONE', #3652, #6789, #10117 ) ;
#6359=ADVANCED_FACE ( 'NONE', ( #8951, #9633 ), #1812, .F. ) ;
#6362=DIRECTION ( 'NONE',  ( 0.000000000000000000, 1.000000000000000000, 0.000000000000000000 ) ) ;
#6412=LINE ( 'NONE', #9589, #6144 ) ;
#6458=LINE ( 'NONE', #6504, #2638 ) ;
#6466=CARTESIAN_POINT ( 'NONE',  ( -166.4201884169622758, -1.620235114669962950, 14.91256936275685341 ) ) ;
#6470=CARTESIAN_POINT ( 'NONE',  ( -164.7175697302053834, 2.136007004543084342, 12.82334789677917364 ) ) ;
#6473=EDGE_LOOP ( 'NONE', ( #311, #2177, #1513, #1663 ) ) ;
#6482=SURFACE_STYLE_FILL_AREA ( #1847 ) ;
#6504=CARTESIAN_POINT ( 'NONE',  ( -8.084771497730057628E-16, 16.99999999999997868, 0.000000000000000000 ) ) ;
#6511=CARTESIAN_POINT ( 'NONE',  ( -163.3797075017903353, -1.420136444163668132, 14.93295499430977991 ) ) ;
#6563=FACE_OUTER_BOUND ( 'NONE', #335, .T. ) ;
#6568=CARTESIAN_POINT ( 'NONE',  ( -167.1500000000000341, -6.071532165918824830E-15, 0.000000000000000000 ) ) ;
#6611=CARTESIAN_POINT ( 'NONE',  ( -167.1500000000000057, 0.1422526577103273016, 15.00000000000000000 ) ) ;
#6644=EDGE_CURVE ( 'NONE', #4085, #3486, #1725, .T. ) ;
#6661=CARTESIAN_POINT ( 'NONE',  ( -164.4418057750100388, 2.081034501115442303, 14.85496774026629119 ) ) ;
#6695=CARTESIAN_POINT ( 'NONE',  ( 9.511495879682431411E-16, -20.00000000000000000, 2.449293598294706513E-15 ) ) ;
#6718=( NAMED_UNIT ( * ) SI_UNIT ( $, .STERADIAN. ) SOLID_ANGLE_UNIT ( ) );
#6738=ORIENTED_EDGE ( 'NONE', *, *, #3324, .T. ) ;
#6754=CARTESIAN_POINT ( 'NONE',  ( -170.0000000000000284, -15.00000000000001066, 1.836970198721029983E-15 ) ) ;
#6760=CARTESIAN_POINT ( 'NONE',  ( -167.1500000000000341, -1.102909754258692077E-14, 15.00000000000000000 ) ) ;
#6776=PRODUCT_DEFINITION_CONTEXT ( 'detailed design', #257, 'design' ) ;
#6789=DIRECTION ( 'NONE',  ( -0.000000000000000000, -0.000000000000000000, -1.000000000000000000 ) ) ;
#6790=DIRECTION ( 'NONE',  ( 1.000000000000000000, 4.755747939841215952E-17, -0.000000000000000000 ) ) ;
#6820=CARTESIAN_POINT ( 'NONE',  ( -167.1360136226436452, -0.2828357332780486177, 12.99766529850317021 ) ) ;
#6823=EDGE_LOOP ( 'NONE', ( #7693, #647 ) ) ;
#6839=EDGE_LOOP ( 'NONE', ( #517, #3989, #6738, #4226 ) ) ;
#6854=FACE_OUTER_BOUND ( 'NONE', #9039, .T. ) ;
#6875=VERTEX_POINT ( 'NONE', #10078 ) ;
#6889=EDGE_LOOP ( 'NONE', ( #1784, #8631, #2921, #8730 ) ) ;
#6950=EDGE_CURVE ( 'NONE', #5716, #8307, #3643, .T. ) ;
#6977=ADVANCED_FACE ( 'NONE', ( #2106, #1330 ), #2925, .F. ) ;
#6980=CARTESIAN_POINT ( 'NONE',  ( -167.1500000000000341, -1.102909754258692077E-14, 15.00000000000000000 ) ) ;
#6998=DIRECTION ( 'NONE',  ( 1.000000000000000000, 4.755747939841215952E-17, -0.000000000000000000 ) ) ;
#7014=EDGE_CURVE ( 'NONE', #8307, #5716, #3987, .T. ) ;
#7037=CARTESIAN_POINT ( 'NONE',  ( -162.8500000000000796, -0.2808225807418253672, 13.00000000000000533 ) ) ;
#7042=CIRCLE ( 'NONE', #3415, 18.00000000000000355 ) ;
#7065=VERTEX_POINT ( 'NONE', #812 ) ;
#7102=AXIS2_PLACEMENT_3D ( 'NONE', #3488, #6001, #2753 ) ;
#7104=VERTEX_POINT ( 'NONE', #4317 ) ;
#7105=EDGE_CURVE ( 'NONE', #7562, #913, #8776, .T. ) ;
#7117=MANIFOLD_SOLID_BREP ( 'M4 Clearance Hole1', #5799 ) ;
#7122=APPLICATION_CONTEXT ( 'automotive_design' ) ;
#7148=ORIENTED_EDGE ( 'NONE', *, *, #9435, .T. ) ;
#7150=DIRECTION ( 'NONE',  ( -4.818676322157796389E-17, 1.000000000000000000, 0.000000000000000000 ) ) ;
#7194=B_SPLINE_CURVE_WITH_KNOTS ( 'NONE', 3,
 ( #6760, #6611, #5185, #9946, #3479, #7405, #4458, #4256, #7558, #8334, #5078, #5843, #8228, #2796, #5945, #6661, #9843, #2081, #1156, #2746, #9125, #5891, #9070, #5229, #1306, #3685, #8178, #9744, #2650, #1979 ),
 .UNSPECIFIED., .F., .F.,
 ( 4, 2, 2, 2, 2, 2, 2, 2, 2, 2, 2, 2, 2, 2, 4 ),
 ( 4.816881890085070803E-18, 0.0004206592251581338219, 0.0008413184503162626565, 0.001261977675474391545, 0.001682636900632520326, 0.002523955350948835566, 0.003365273801265151240, 0.003785933026423350060, 0.004206592251581550181, 0.004627251476739749000, 0.005047910701897948688, 0.005468569927056148375, 0.005889229152214347195, 0.006309888377372546882, 0.006730547602530746569 ),
 .UNSPECIFIED. ) ;
#7227=CARTESIAN_POINT ( 'NONE',  ( -158.0000000000000284, -18.00000000000001066, 2.204364238465236217E-15 ) ) ;
#7234=ADVANCED_FACE ( 'NONE', ( #2809, #291 ), #2038, .T. ) ;
#7253=CARTESIAN_POINT ( 'NONE',  ( -167.1500000000000341, -5.483569848023176209E-15, 13.00000000000000178 ) ) ;
#7281=AXIS2_PLACEMENT_3D ( 'NONE', #4343, #9007, #1918 ) ;
#7306=CARTESIAN_POINT ( 'NONE',  ( -167.0812335317077668, 0.5573535649547497473, 12.98877602732082615 ) ) ;
#7316=CARTESIAN_POINT ( 'NONE',  ( -158.0000000000000284, 14.99999999999999289, 0.000000000000000000 ) ) ;
#7319=UNCERTAINTY_MEASURE_WITH_UNIT (LENGTH_MEASURE( 1.000000000000000082E-05 ), #1172, 'distance_accuracy_value', 'NONE');
#7329=ORIENTED_EDGE ( 'NONE', *, *, #755, .T. ) ;
#7350=CARTESIAN_POINT ( 'NONE',  ( -2.000000000000001776, -9.511495879682425741E-17, 0.000000000000000000 ) ) ;
#7354=CARTESIAN_POINT ( 'NONE',  ( -167.1500000000000057, -0.2844360088669644626, 15.00000000000000000 ) ) ;
#7391=ORIENTED_EDGE ( 'NONE', *, *, #3324, .F. ) ;
#7402=CARTESIAN_POINT ( 'NONE',  ( -163.9214193032601656, -1.865165441064630780, 14.88379409306876866 ) ) ;
#7405=CARTESIAN_POINT ( 'NONE',  ( -166.9318441561673012, 0.9541142454723345878, 14.97019227849299128 ) ) ;
#7409=ORIENTED_EDGE ( 'NONE', *, *, #6644, .T. ) ;
#7419=DIRECTION ( 'NONE',  ( 1.000000000000000000, 0.000000000000000000, 0.000000000000000000 ) ) ;
#7426=ORIENTED_EDGE ( 'NONE', *, *, #2922, .T. ) ;
#7434=AXIS2_PLACEMENT_3D ( 'NONE', #8506, #8662, #7830 ) ;
#7491=CARTESIAN_POINT ( 'NONE',  ( -158.0000000000000284, -7.514081744949122117E-15, 0.000000000000000000 ) ) ;
#7532=ORIENTED_EDGE ( 'NONE', *, *, #5402, .T. ) ;
#7546=DIRECTION ( 'NONE',  ( -4.755747939841216568E-17, 1.000000000000000000, 0.000000000000000000 ) ) ;
#7558=CARTESIAN_POINT ( 'NONE',  ( -166.6190172193898036, 1.421584020712995056, 14.93281639362370328 ) ) ;
#7562=VERTEX_POINT ( 'NONE', #5295 ) ;
#7617=ADVANCED_FACE ( 'NONE', ( #3857 ), #3953, .F. ) ;
#7624=LINE ( 'NONE', #8107, #386 ) ;
#7634=EDGE_CURVE ( 'NONE', #3486, #4085, #5453, .T. ) ;
#7641=DIRECTION ( 'NONE',  ( -4.755747939841215952E-17, 1.000000000000000000, 0.000000000000000000 ) ) ;
#7649=ORIENTED_EDGE ( 'NONE', *, *, #6950, .T. ) ;
#7664=EDGE_LOOP ( 'NONE', ( #5282, #7391 ) ) ;
#7678=ORIENTED_EDGE ( 'NONE', *, *, #6058, .T. ) ;
#7687=CARTESIAN_POINT ( 'NONE',  ( 0.000000000000000000, 0.000000000000000000, 0.000000000000000000 ) ) ;
#7693=ORIENTED_EDGE ( 'NONE', *, *, #2537, .T. ) ;
#7704=EDGE_LOOP ( 'NONE', ( #1707, #2158 ) ) ;
#7705=FACE_BOUND ( 'NONE', #261, .T. ) ;
#7719=DIRECTION ( 'NONE',  ( -1.000000000000000000, -4.755747939841215952E-17, 0.000000000000000000 ) ) ;
#7724=CARTESIAN_POINT ( 'NONE',  ( -166.7172248328349724, -1.323598984370104814, 12.93397516672917646 ) ) ;
#7733=DIRECTION ( 'NONE',  ( 1.000000000000000000, 4.755747939841215952E-17, -0.000000000000000000 ) ) ;
#7773=AXIS2_PLACEMENT_3D ( 'NONE', #4617, #5339, #3846 ) ;
#7819=CARTESIAN_POINT ( 'NONE',  ( -164.0445443052358314, -1.931192361225922971, 12.85587404590432392 ) ) ;
#7830=DIRECTION ( 'NONE',  ( 0.000000000000000000, 1.000000000000000000, 0.000000000000000000 ) ) ;
#7853=ADVANCED_FACE ( 'NONE', ( #5398 ), #3905, .T. ) ;
#7865=CARTESIAN_POINT ( 'NONE',  ( -165.2805265249035074, -2.136232373723711664, 12.82330986584687693 ) ) ;
#7873=CARTESIAN_POINT ( 'NONE',  ( -170.0000000000000284, -8.084771497730068080E-15, 0.000000000000000000 ) ) ;
#7878=DIRECTION ( 'NONE',  ( 1.000000000000000000, 4.755747939841215952E-17, -0.000000000000000000 ) ) ;
#7932=VECTOR ( 'NONE', #714, 1000.000000000000000 ) ;
#7953=EDGE_LOOP ( 'NONE', ( #5415, #7148, #1565, #1345 ) ) ;
#7973=EDGE_CURVE ( 'NONE', #1436, #8355, #2381, .T. ) ;
#7975=CIRCLE ( 'NONE', #9800, 16.99999999999997868 ) ;
#7982=CARTESIAN_POINT ( 'NONE',  ( -163.2908618794298832, 1.311844299765515753, 12.93416838467167196 ) ) ;
#7998=CARTESIAN_POINT ( 'NONE',  ( -167.1500000000000341, -5.483569848023176209E-15, 13.00000000000000178 ) ) ;
#8000=ORIENTED_EDGE ( 'NONE', *, *, #3345, .F. ) ;
#8002=CARTESIAN_POINT ( 'NONE',  ( -158.0000000000000284, 12.99999999999999289, 0.000000000000000000 ) ) ;
#8067=EDGE_CURVE ( 'NONE', #5081, #2751, #679, .T. ) ;
#8079=CARTESIAN_POINT ( 'NONE',  ( -163.0677828165198662, 0.9533406220131400710, 12.96565173575652175 ) ) ;
#8088=ADVANCED_FACE ( 'NONE', ( #6563 ), #2402, .F. ) ;
#8107=CARTESIAN_POINT ( 'NONE',  ( 6.182472321793581601E-16, -13.00000000000000178, 1.592040838891559293E-15 ) ) ;
#8122=DIRECTION ( 'NONE',  ( 1.000000000000000000, 4.755747939841215952E-17, -0.000000000000000000 ) ) ;
#8127=CARTESIAN_POINT ( 'NONE',  ( -165.6923089559685138, -2.040351103243558395, 14.86068369067391792 ) ) ;
#8133=ORIENTED_EDGE ( 'NONE', *, *, #2093, .T. ) ;
#8178=CARTESIAN_POINT ( 'NONE',  ( -162.9191712434781039, 0.5589657928192890424, 14.99021695762547424 ) ) ;
#8210=EDGE_CURVE ( 'NONE', #7104, #8355, #8974, .T. ) ;
#8228=CARTESIAN_POINT ( 'NONE',  ( -165.2816655742341823, 2.149895177073305685, 14.84513222368812002 ) ) ;
#8235=CYLINDRICAL_SURFACE ( 'NONE', #2802, 20.00000000000000000 ) ;
#8237=DIRECTION ( 'NONE',  ( 1.000000000000000000, 4.755747939841215952E-17, -0.000000000000000000 ) ) ;
#8243=EDGE_CURVE ( 'NONE', #6156, #7104, #7194, .T. ) ;
#8244=( NAMED_UNIT ( * ) PLANE_ANGLE_UNIT ( ) SI_UNIT ( $, .RADIAN. ) );
#8271=DIRECTION ( 'NONE',  ( 1.000000000000000000, 4.755747939841215952E-17, -0.000000000000000000 ) ) ;
#8288=ORIENTED_EDGE ( 'NONE', *, *, #8067, .T. ) ;
#8294=EDGE_CURVE ( 'NONE', #6875, #4862, #3971, .T. ) ;
#8301=DIRECTION ( 'NONE',  ( -4.755747939841215952E-17, 1.000000000000000000, 0.000000000000000000 ) ) ;
#8307=VERTEX_POINT ( 'NONE', #1885 ) ;
#8334=CARTESIAN_POINT ( 'NONE',  ( -166.3218336876412593, 1.718641102943201604, 14.90254673046750433 ) ) ;
#8355=VERTEX_POINT ( 'NONE', #9994 ) ;
#8419=AXIS2_PLACEMENT_3D ( 'NONE', #4108, #1631, #4009 ) ;
#8426=COLOUR_RGB ( '', 0.72549020, 0.75294118, 0.79215686) ;
#8440=CARTESIAN_POINT ( 'NONE',  ( -163.6882088544006706, -1.709196472000179323, 12.88739062898286214 ) ) ;
#8453=VECTOR ( 'NONE', #1754, 1000.000000000000000 ) ;
#8461=EDGE_LOOP ( 'NONE', ( #1760, #3963 ) ) ;
#8490=DIRECTION ( 'NONE',  ( 1.000000000000000000, 4.755747939841215952E-17, -0.000000000000000000 ) ) ;
#8506=CARTESIAN_POINT ( 'NONE',  ( -158.0000000000000284, -7.514081744949122117E-15, 0.000000000000000000 ) ) ;
#8517=EDGE_CURVE ( 'NONE', #8355, #1436, #4600, .T. ) ;
#8540=EDGE_CURVE ( 'NONE', #6270, #7065, #10077, .T. ) ;
#8542=AXIS2_PLACEMENT_3D ( 'NONE', #4602, #10075, #6234 ) ;
#8545=CARTESIAN_POINT ( 'NONE',  ( -164.3050676404916715, -2.039477515547296171, 12.83914065986469488 ) ) ;
#8563=ORIENTED_EDGE ( 'NONE', *, *, #8294, .T. ) ;
#8591=PLANE ( 'NONE',  #3676 ) ;
#8610=ADVANCED_FACE ( 'NONE', ( #3059, #6203 ), #8902, .T. ) ;
#8631=ORIENTED_EDGE ( 'NONE', *, *, #8210, .T. ) ;
#8650=CARTESIAN_POINT ( 'NONE',  ( -162.9065109726407456, -0.5641505380384801427, 12.99034143968891541 ) ) ;
#8659=CARTESIAN_POINT ( 'NONE',  ( -160.0000000000000284, -15.00000000000000711, 1.836970198721029589E-15 ) ) ;
#8662=DIRECTION ( 'NONE',  ( 1.000000000000000000, 4.755747939841215952E-17, -0.000000000000000000 ) ) ;
#8668=CYLINDRICAL_SURFACE ( 'NONE', #675, 16.99999999999997868 ) ;
#8680=ORIENTED_EDGE ( 'NONE', *, *, #8067, .F. ) ;
#8698=EDGE_CURVE ( 'NONE', #8824, #6875, #5539, .T. ) ;
#8699=CARTESIAN_POINT ( 'NONE',  ( -2.000000000000001776, 20.00000000000000000, 0.000000000000000000 ) ) ;
#8709=CARTESIAN_POINT ( 'NONE',  ( -163.9213440228380989, 1.865096155104054354, 12.86575230306539908 ) ) ;
#8711=DIRECTION ( 'NONE',  ( 1.000000000000000000, 4.755747939841215952E-17, -0.000000000000000000 ) ) ;
#8730=ORIENTED_EDGE ( 'NONE', *, *, #2171, .F. ) ;
#8744=DIRECTION ( 'NONE',  ( -4.755747939841215952E-17, 1.000000000000000000, 0.000000000000000000 ) ) ;
#8759=CARTESIAN_POINT ( 'NONE',  ( -167.1500000000000341, 0.1423186749851698130, 13.00000000000000000 ) ) ;
#8769=CARTESIAN_POINT ( 'NONE',  ( 0.000000000000000000, 0.000000000000000000, 0.000000000000000000 ) ) ;
#8776=CIRCLE ( 'NONE', #1341, 20.00000000000000000 ) ;
#8808=CARTESIAN_POINT ( 'NONE',  ( -158.0000000000000284, 17.99999999999999645, 0.000000000000000000 ) ) ;
#8817=DIRECTION ( 'NONE',  ( 1.000000000000000000, 4.755747939841215952E-17, -0.000000000000000000 ) ) ;
#8820=CARTESIAN_POINT ( 'NONE',  ( -167.0397669596979426, 0.6940490614466876540, 12.98211462413728157 ) ) ;
#8824=VERTEX_POINT ( 'NONE', #8808 ) ;
#8841=EDGE_LOOP ( 'NONE', ( #1472, #5207 ) ) ;
#8857=CARTESIAN_POINT ( 'NONE',  ( -8.560346291714190440E-16, 18.00000000000000355, 0.000000000000000000 ) ) ;
#8866=DIRECTION ( 'NONE',  ( 1.000000000000000000, 4.755747939841215952E-17, -0.000000000000000000 ) ) ;
#8898=CARTESIAN_POINT ( 'NONE',  ( 0.000000000000000000, 0.000000000000000000, 0.000000000000000000 ) ) ;
#8902=PLANE ( 'NONE',  #6267 ) ;
#8910=CARTESIAN_POINT ( 'NONE',  ( -163.0672239440268356, -0.9520965995333376952, 14.97031403060969446 ) ) ;
#8913=CARTESIAN_POINT ( 'NONE',  ( -162.8500000000000796, 0.1404462806920659668, 13.00000000000000533 ) ) ;
#8922=SURFACE_SIDE_STYLE ('',( #1989 ) ) ;
#8930=DIRECTION ( 'NONE',  ( 0.000000000000000000, 0.000000000000000000, 1.000000000000000000 ) ) ;
#8948=MECHANICAL_DESIGN_GEOMETRIC_PRESENTATION_REPRESENTATION('',(#5948),#1680);
#8951=FACE_OUTER_BOUND ( 'NONE', #2074, .T. ) ;
#8955=AXIS2_PLACEMENT_3D ( 'NONE', #4364, #1987, #10049 ) ;
#8969=CARTESIAN_POINT ( 'NONE',  ( -164.7164049854163181, -2.135816869796272943, 14.84719012526269388 ) ) ;
#8974=LINE ( 'NONE', #434, #5775 ) ;
#8987=( NAMED_UNIT ( * ) PLANE_ANGLE_UNIT ( ) SI_UNIT ( $, .RADIAN. ) );
#9007=DIRECTION ( 'NONE',  ( 1.000000000000000000, 4.755747939841215952E-17, -0.000000000000000000 ) ) ;
#9010=EDGE_CURVE ( 'NONE', #557, #3401, #6458, .T. ) ;
#9039=EDGE_LOOP ( 'NONE', ( #2532, #4329, #5140, #1451 ) ) ;
#9070=CARTESIAN_POINT ( 'NONE',  ( -163.2907867177267462, 1.311749039217684709, 14.94298962415842880 ) ) ;
#9078=DIRECTION ( 'NONE',  ( 0.000000000000000000, 1.000000000000000000, 0.000000000000000000 ) ) ;
#9113=ADVANCED_FACE ( 'NONE', ( #9937 ), #9880, .F. ) ;
#9125=CARTESIAN_POINT ( 'NONE',  ( -163.5800396265123595, 1.620586088255114188, 14.91253992662286976 ) ) ;
#9129=ORIENTED_EDGE ( 'NONE', *, *, #9774, .T. ) ;
#9157=EDGE_CURVE ( 'NONE', #913, #7562, #4478, .T. ) ;
#9206=FACE_OUTER_BOUND ( 'NONE', #3714, .T. ) ;
#9278=CARTESIAN_POINT ( 'NONE',  ( -165.9526703272678958, -1.932542173981024458, 12.85566991495389466 ) ) ;
#9284=EDGE_CURVE ( 'NONE', #1035, #557, #4643, .T. ) ;
#9287=FACE_BOUND ( 'NONE', #2507, .T. ) ;
#9311=DIRECTION ( 'NONE',  ( -1.000000000000000000, 0.000000000000000000, 0.000000000000000000 ) ) ;
#9346=LINE ( 'NONE', #3962, #7932 ) ;
#9369=CIRCLE ( 'NONE', #3911, 15.00000000000000000 ) ;
#9378=CARTESIAN_POINT ( 'NONE',  ( -162.8500000000000512, -5.808233196467851957E-15, 13.00000000000000178 ) ) ;
#9409=VERTEX_POINT ( 'NONE', #6695 ) ;
#9411=CYLINDRICAL_SURFACE ( 'NONE', #2268, 2.149999999999985256 ) ;
#9421=AXIS2_PLACEMENT_3D ( 'NONE', #1586, #8711, #3124 ) ;
#9425=FACE_OUTER_BOUND ( 'NONE', #6823, .T. ) ;
#9431=CARTESIAN_POINT ( 'NONE',  ( -165.5557670730357529, -2.081659637464541301, 12.83228186348094901 ) ) ;
#9435=EDGE_CURVE ( 'NONE', #7562, #9409, #9787, .T. ) ;
#9488=ORIENTED_EDGE ( 'NONE', *, *, #9010, .F. ) ;
#9517=EDGE_LOOP ( 'NONE', ( #5644, #715, #7532, #6035 ) ) ;
#9540=DIRECTION ( 'NONE',  ( -4.755747939841215952E-17, 1.000000000000000000, 0.000000000000000000 ) ) ;
#9543=CARTESIAN_POINT ( 'NONE',  ( -167.1360087209127130, 0.2822104782917173038, 12.99766528766663853 ) ) ;
#9574=ORIENTED_EDGE ( 'NONE', *, *, #1343, .T. ) ;
#9589=CARTESIAN_POINT ( 'NONE',  ( -9.511495879682431411E-16, 20.00000000000000000, 0.000000000000000000 ) ) ;
#9603=EDGE_LOOP ( 'NONE', ( #3454, #7649, #8133, #8680 ) ) ;
#9622=ORIENTED_EDGE ( 'NONE', *, *, #4219, .T. ) ;
#9633=FACE_BOUND ( 'NONE', #664, .T. ) ;
#9637=DIRECTION ( 'NONE',  ( 4.755747939841215952E-17, -1.000000000000000000, 0.000000000000000000 ) ) ;
#9644=DIRECTION ( 'NONE',  ( 1.000000000000000000, 4.755747939841215952E-17, -0.000000000000000000 ) ) ;
#9645=CARTESIAN_POINT ( 'NONE',  ( -163.5777460020251795, -1.618434078064680870, 14.91276646089121627 ) ) ;
#9648=CARTESIAN_POINT ( 'NONE',  ( -164.4416275561781333, 2.080988465785847286, 12.83239121171710018 ) ) ;
#9661=( LENGTH_UNIT ( ) NAMED_UNIT ( * ) SI_UNIT ( .MILLI., .METRE. ) );
#9686=ADVANCED_BREP_SHAPE_REPRESENTATION ( '', ( #7117, #3995 ), #10094 ) ;
#9693=CARTESIAN_POINT ( 'NONE',  ( -162.9599602851104976, 0.6932240239557875272, 12.98215789948331889 ) ) ;
#9707=CYLINDRICAL_SURFACE ( 'NONE', #1180, 15.00000000000000000 ) ;
#9730=CARTESIAN_POINT ( 'NONE',  ( -170.0000000000000284, 12.99999999999999289, 0.000000000000000000 ) ) ;
#9744=CARTESIAN_POINT ( 'NONE',  ( -162.8640756141387840, 0.2830513900230973712, 14.99796416534026200 ) ) ;
#9752=AXIS2_PLACEMENT_3D ( 'NONE', #4356, #5798, #1252 ) ;
#9754=PRESENTATION_STYLE_ASSIGNMENT (( #3434 ) ) ;
#9762=PRESENTATION_STYLE_ASSIGNMENT (( #4220 ) ) ;
#9774=EDGE_CURVE ( 'NONE', #1035, #5632, #10185, .T. ) ;
#9787=LINE ( 'NONE', #2689, #5624 ) ;
#9800=AXIS2_PLACEMENT_3D ( 'NONE', #3402, #3118, #6259 ) ;
#9812=( NAMED_UNIT ( * ) SI_UNIT ( $, .STERADIAN. ) SOLID_ANGLE_UNIT ( ) );
#9843=CARTESIAN_POINT ( 'NONE',  ( -164.3076905434401453, 2.040364482056596707, 14.86068217355785670 ) ) ;
#9847=ORIENTED_EDGE ( 'NONE', *, *, #8243, .T. ) ;
#9851=FILL_AREA_STYLE_COLOUR ( '', #8426 ) ;
#9880=CYLINDRICAL_SURFACE ( 'NONE', #10086, 16.99999999999997868 ) ;
#9918=CYLINDRICAL_SURFACE ( 'NONE', #6291, 2.149999999999985256 ) ;
#9937=FACE_OUTER_BOUND ( 'NONE', #1400, .T. ) ;
#9946=CARTESIAN_POINT ( 'NONE',  ( -167.0812848797259562, 0.5571504444270253265, 14.99028060246901006 ) ) ;
#9994=CARTESIAN_POINT ( 'NONE',  ( -162.8500000000000512, -5.808233196467851957E-15, 13.00000000000000178 ) ) ;
#10032=DIRECTION ( 'NONE',  ( 1.000000000000000000, 4.755747939841215952E-17, -0.000000000000000000 ) ) ;
#10041=CARTESIAN_POINT ( 'NONE',  ( -163.5777872869976761, -1.618470104113066910, 12.89924494662433396 ) ) ;
#10049=DIRECTION ( 'NONE',  ( 0.000000000000000000, 1.000000000000000000, 0.000000000000000000 ) ) ;
#10075=DIRECTION ( 'NONE',  ( 1.000000000000000000, 4.755747939841215952E-17, -0.000000000000000000 ) ) ;
#10077=CIRCLE ( 'NONE', #7773, 13.00000000000000178 ) ;
#10078=CARTESIAN_POINT ( 'NONE',  ( -2.000000000000002665, 18.00000000000000355, 0.000000000000000000 ) ) ;
#10086=AXIS2_PLACEMENT_3D ( 'NONE', #2784, #8271, #7546 ) ;
#10094=( GEOMETRIC_REPRESENTATION_CONTEXT ( 3 ) GLOBAL_UNCERTAINTY_ASSIGNED_CONTEXT ( ( #2041 ) ) GLOBAL_UNIT_ASSIGNED_CONTEXT ( ( #9661, #8244, #9812 ) ) REPRESENTATION_CONTEXT ( 'NONE', 'WORKASPACE' ) );
#10106=LINE ( 'NONE', #4625, #890 ) ;
#10107=FACE_OUTER_BOUND ( 'NONE', #6473, .T. ) ;
#10111=DIRECTION ( 'NONE',  ( -4.755747939841215952E-17, 1.000000000000000000, 0.000000000000000000 ) ) ;
#10117=DIRECTION ( 'NONE',  ( -1.000000000000000000, 0.000000000000000000, 0.000000000000000000 ) ) ;
#10124=ORIENTED_EDGE ( 'NONE', *, *, #6950, .F. ) ;
#10185=LINE ( 'NONE', #6192, #4145 ) ;
#10205=CARTESIAN_POINT ( 'NONE',  ( -9.511495879682431411E-16, 20.00000000000000000, 0.000000000000000000 ) ) ;
#10214=ADVANCED_FACE ( 'NONE', ( #5151 ), #9707, .T. ) ;
ENDSEC;
END-ISO-10303-21;
